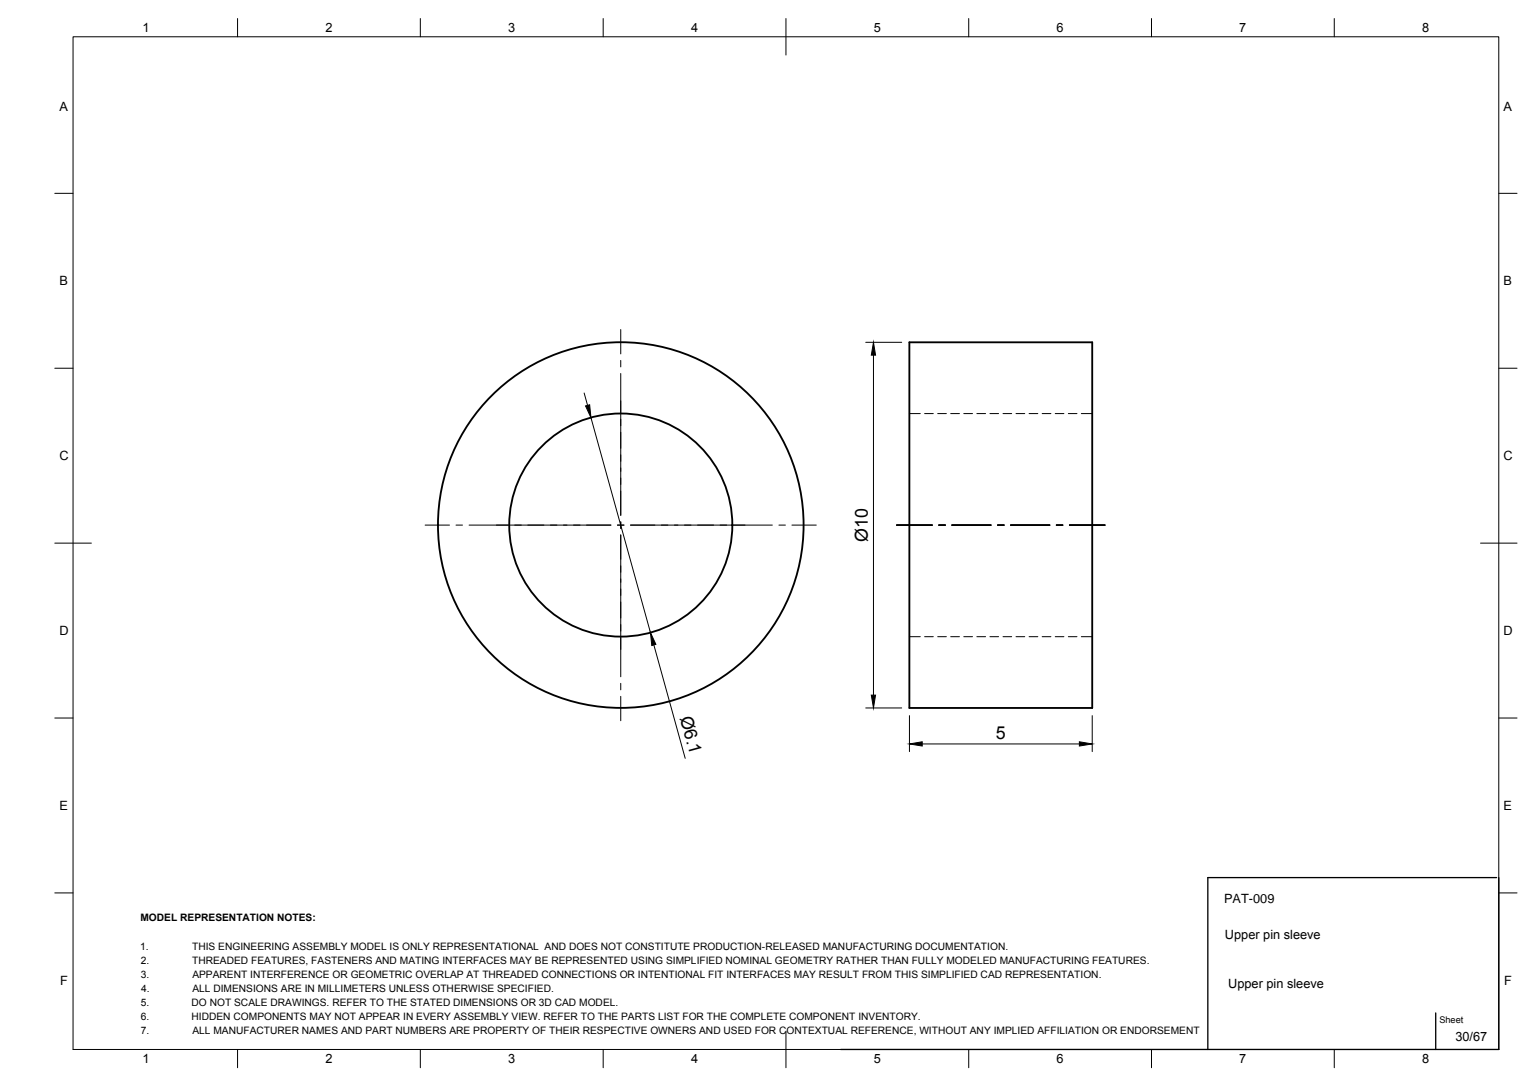
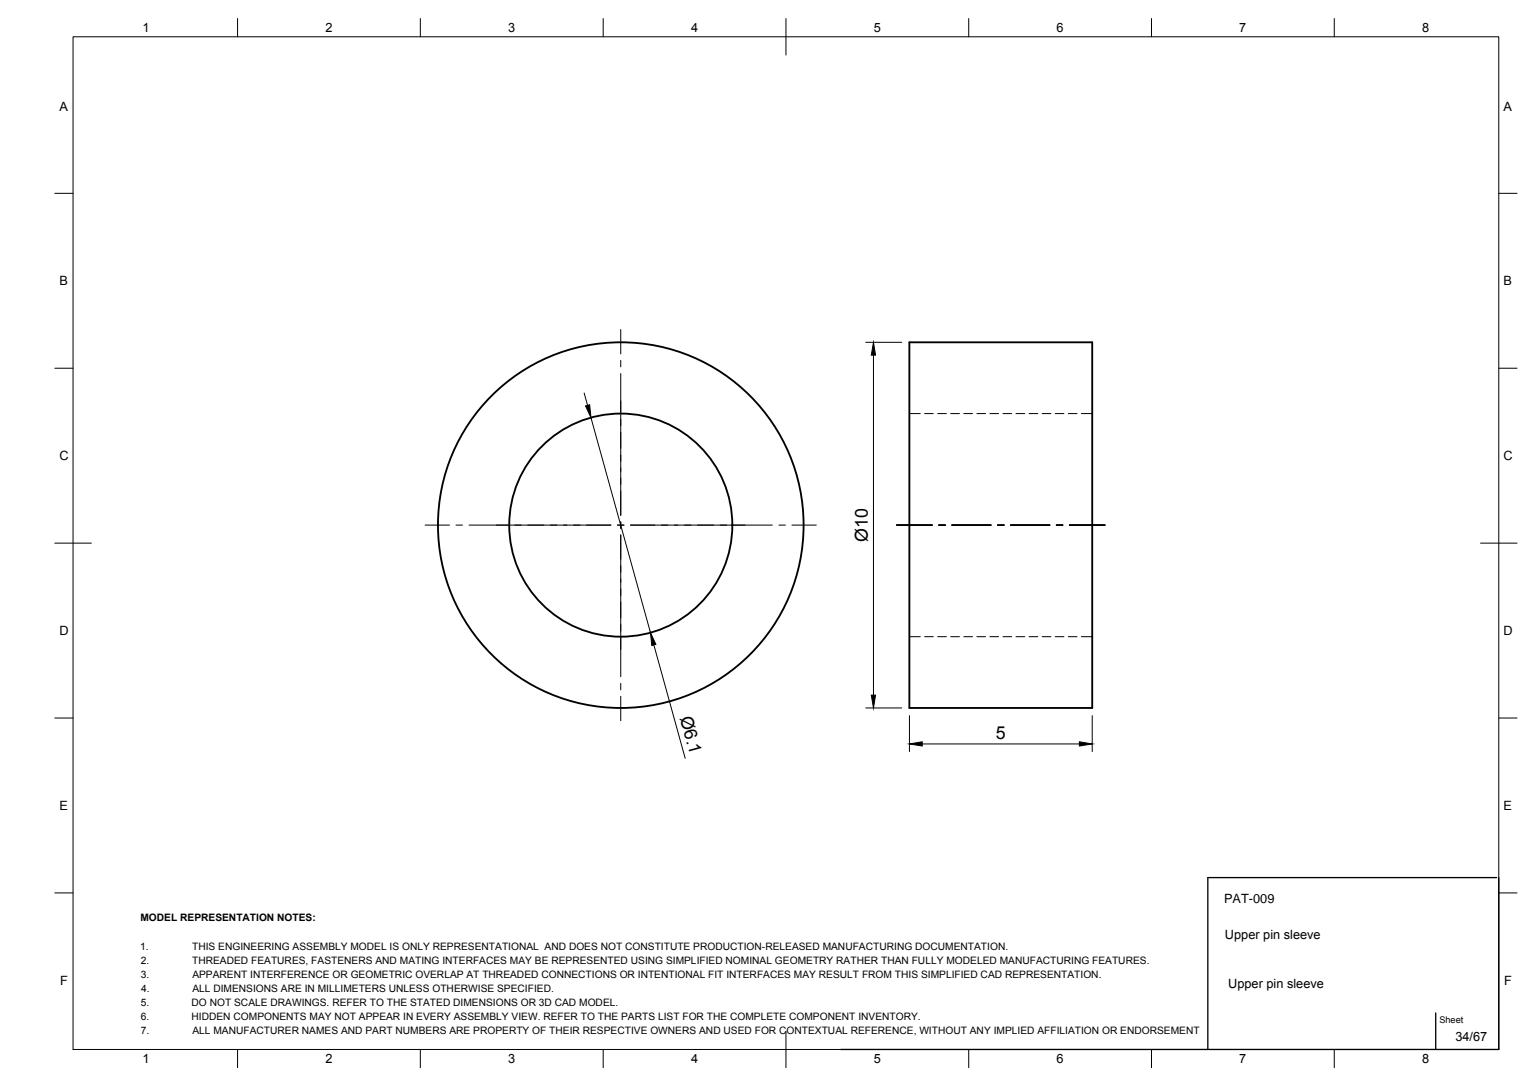
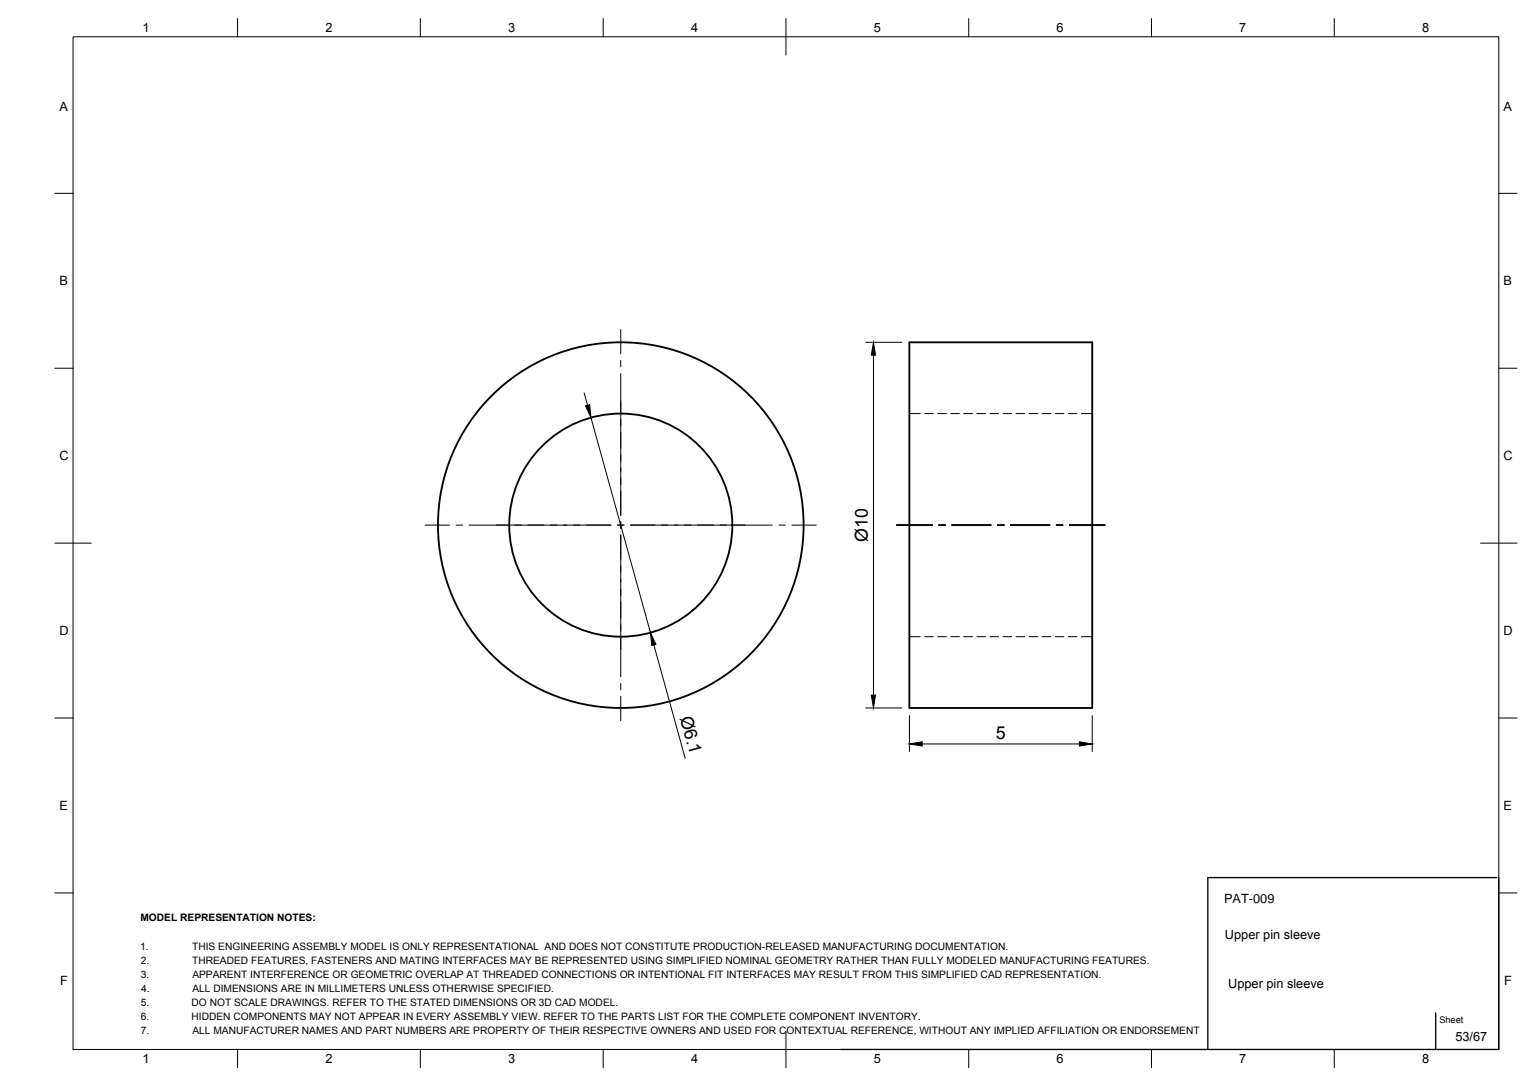
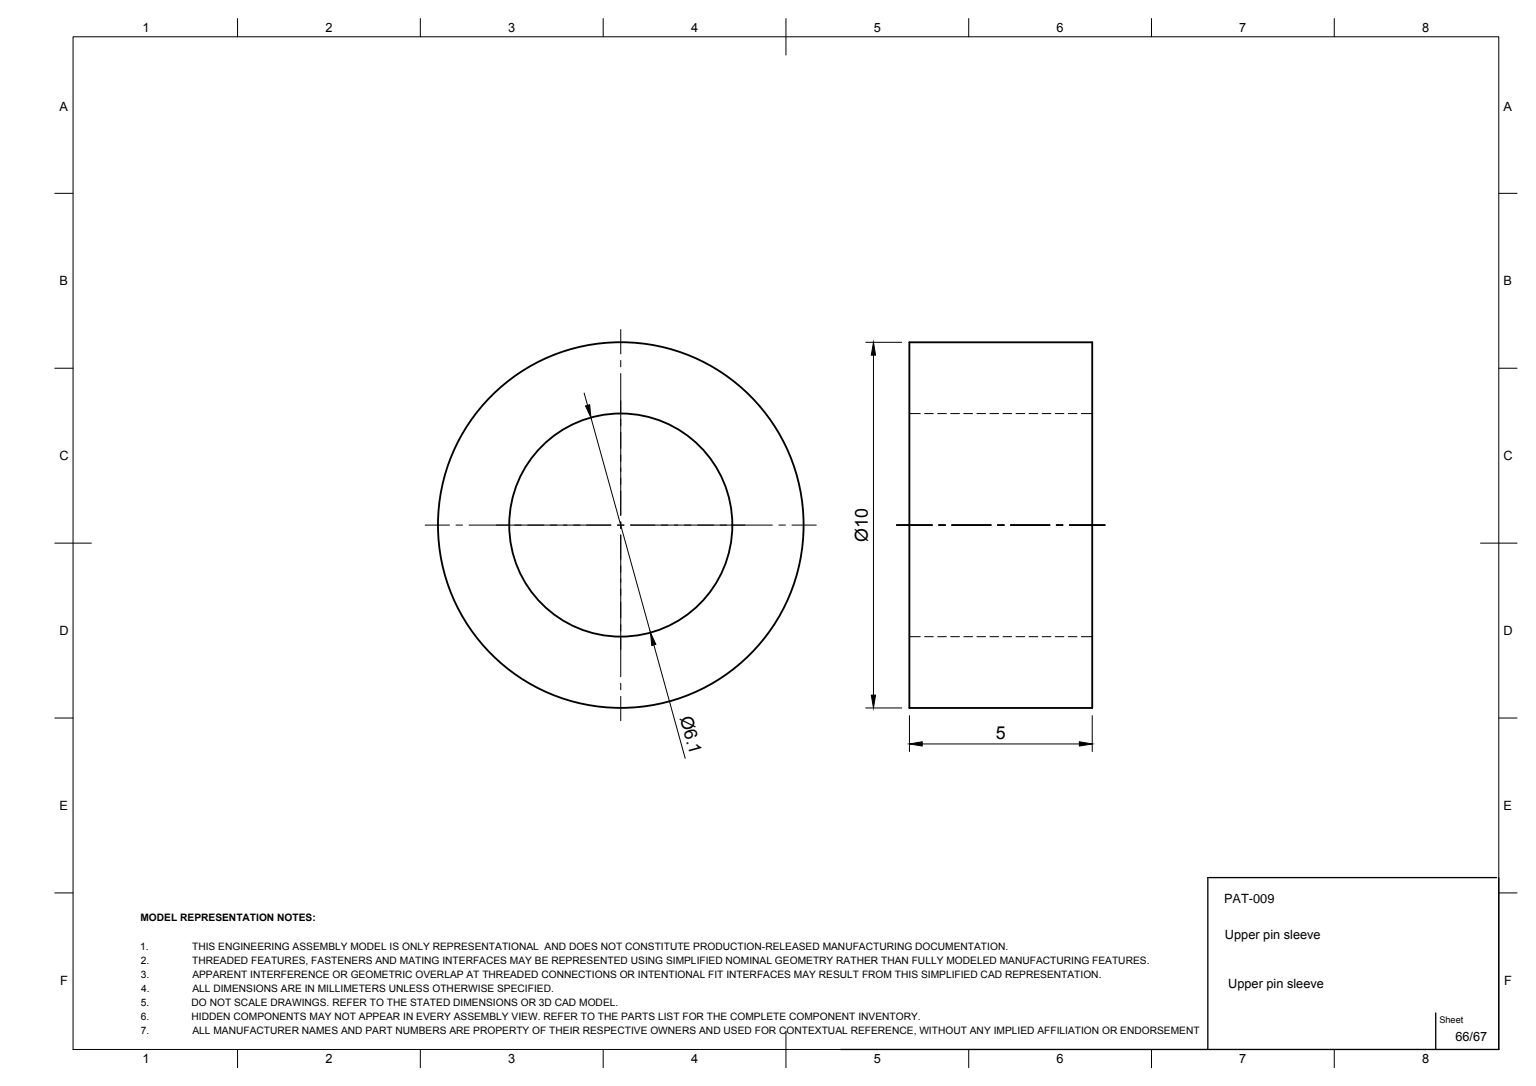
ISO-10303-21;
HEADER;
/* Generated by software containing ST-Developer
 * from STEP Tools, Inc. (www.steptools.com) 
 */

FILE_DESCRIPTION(
/* description */ ('Bell-crank linkage with push rods'),
/* implementation_level */ '2;1');

FILE_NAME(
/* name */ 'Upper pin sleeve.step',
/* time_stamp */ '2026-10-28T03:25:15-07:00',
/* author */ (''),
/* organization */ (''),
/* preprocessor_version */ 'ST-DEVELOPER v20.2',
/* originating_system */ 'Autodesk Translation Framework v15.17.0.0',
/* authorisation */ '');

FILE_SCHEMA (('AUTOMOTIVE_DESIGN { 1 0 10303 214 3 1 1 }'));
ENDSEC;

DATA;
#10=MECHANICAL_DESIGN_GEOMETRIC_PRESENTATION_REPRESENTATION('',(#635),#16678);
#519=SHAPE_REPRESENTATION_RELATIONSHIP('SRR','None',#16937,#573);
#573=ADVANCED_BREP_SHAPE_REPRESENTATION('',(#696),#16642);
#635=STYLED_ITEM('',(#17291),#696);
#696=MANIFOLD_SOLID_BREP('Body1',#8826);
#843=FACE_BOUND('',#2170,.T.);
#844=FACE_BOUND('',#2172,.T.);
#1108=PLANE('',#10059);
#1109=PLANE('',#10060);
#1527=FACE_OUTER_BOUND('',#2167,.T.);
#1528=FACE_OUTER_BOUND('',#2168,.T.);
#1529=FACE_OUTER_BOUND('',#2169,.T.);
#1530=FACE_OUTER_BOUND('',#2171,.T.);
#2167=EDGE_LOOP('',(#7141,#7142,#7143,#7144));
#2168=EDGE_LOOP('',(#7145,#7146,#7147,#7148));
#2169=EDGE_LOOP('',(#7149));
#2170=EDGE_LOOP('',(#7150));
#2171=EDGE_LOOP('',(#7151));
#2172=EDGE_LOOP('',(#7152));
#2822=LINE('',#15413,#3371);
#2823=LINE('',#15419,#3372);
#3371=VECTOR('',#12122,0.305);
#3372=VECTOR('',#12129,0.5);
#3916=CIRCLE('',#10054,0.305);
#3917=CIRCLE('',#10055,0.305);
#3918=CIRCLE('',#10057,0.5);
#3919=CIRCLE('',#10058,0.5);
#4527=VERTEX_POINT('',#15410);
#4528=VERTEX_POINT('',#15412);
#4529=VERTEX_POINT('',#15416);
#4530=VERTEX_POINT('',#15418);
#5448=EDGE_CURVE('',#4527,#4527,#3916,.T.);
#5449=EDGE_CURVE('',#4527,#4528,#2822,.T.);
#5450=EDGE_CURVE('',#4528,#4528,#3917,.T.);
#5451=EDGE_CURVE('',#4529,#4529,#3918,.T.);
#5452=EDGE_CURVE('',#4529,#4530,#2823,.T.);
#5453=EDGE_CURVE('',#4530,#4530,#3919,.T.);
#7141=ORIENTED_EDGE('',*,*,#5448,.F.);
#7142=ORIENTED_EDGE('',*,*,#5449,.T.);
#7143=ORIENTED_EDGE('',*,*,#5450,.T.);
#7144=ORIENTED_EDGE('',*,*,#5449,.F.);
#7145=ORIENTED_EDGE('',*,*,#5451,.F.);
#7146=ORIENTED_EDGE('',*,*,#5452,.T.);
#7147=ORIENTED_EDGE('',*,*,#5453,.T.);
#7148=ORIENTED_EDGE('',*,*,#5452,.F.);
#7149=ORIENTED_EDGE('',*,*,#5451,.T.);
#7150=ORIENTED_EDGE('',*,*,#5448,.T.);
#7151=ORIENTED_EDGE('',*,*,#5453,.F.);
#7152=ORIENTED_EDGE('',*,*,#5450,.F.);
#8177=CYLINDRICAL_SURFACE('',#10053,0.305);
#8178=CYLINDRICAL_SURFACE('',#10056,0.5);
#8552=ADVANCED_FACE('',(#1527),#8177,.F.);
#8553=ADVANCED_FACE('',(#1528),#8178,.T.);
#8554=ADVANCED_FACE('',(#1529,#843),#1108,.T.);
#8555=ADVANCED_FACE('',(#1530,#844),#1109,.F.);
#8826=CLOSED_SHELL('',(#8552,#8553,#8554,#8555));
#10052=AXIS2_PLACEMENT_3D('',#15408,#12116,#12117);
#10053=AXIS2_PLACEMENT_3D('',#15409,#12118,#12119);
#10054=AXIS2_PLACEMENT_3D('',#15411,#12120,#12121);
#10055=AXIS2_PLACEMENT_3D('',#15414,#12123,#12124);
#10056=AXIS2_PLACEMENT_3D('',#15415,#12125,#12126);
#10057=AXIS2_PLACEMENT_3D('',#15417,#12127,#12128);
#10058=AXIS2_PLACEMENT_3D('',#15420,#12130,#12131);
#10059=AXIS2_PLACEMENT_3D('',#15421,#12132,#12133);
#10060=AXIS2_PLACEMENT_3D('',#15422,#12134,#12135);
#12116=DIRECTION('axis',(0.,0.,1.));
#12117=DIRECTION('refdir',(1.,0.,0.));
#12118=DIRECTION('center_axis',(0.,0.,1.));
#12119=DIRECTION('ref_axis',(1.,0.,0.));
#12120=DIRECTION('center_axis',(0.,0.,-1.));
#12121=DIRECTION('ref_axis',(1.,0.,0.));
#12122=DIRECTION('',(0.,0.,-1.));
#12123=DIRECTION('center_axis',(0.,0.,-1.));
#12124=DIRECTION('ref_axis',(1.,0.,0.));
#12125=DIRECTION('center_axis',(0.,0.,1.));
#12126=DIRECTION('ref_axis',(1.,0.,0.));
#12127=DIRECTION('center_axis',(0.,0.,1.));
#12128=DIRECTION('ref_axis',(1.,0.,0.));
#12129=DIRECTION('',(0.,0.,-1.));
#12130=DIRECTION('center_axis',(0.,0.,1.));
#12131=DIRECTION('ref_axis',(1.,0.,0.));
#12132=DIRECTION('center_axis',(0.,0.,1.));
#12133=DIRECTION('ref_axis',(1.,0.,0.));
#12134=DIRECTION('center_axis',(0.,0.,1.));
#12135=DIRECTION('ref_axis',(1.,0.,0.));
#15408=CARTESIAN_POINT('',(0.,0.,0.));
#15409=CARTESIAN_POINT('Origin',(0.,2.,9.6));
#15410=CARTESIAN_POINT('',(-0.305,2.,10.1));
#15411=CARTESIAN_POINT('Origin',(0.,2.,10.1));
#15412=CARTESIAN_POINT('',(-0.305,2.,9.6));
#15413=CARTESIAN_POINT('',(-0.305,2.,9.6));
#15414=CARTESIAN_POINT('Origin',(0.,2.,9.6));
#15415=CARTESIAN_POINT('Origin',(0.,2.,9.6));
#15416=CARTESIAN_POINT('',(-0.5,2.,10.1));
#15417=CARTESIAN_POINT('Origin',(0.,2.,10.1));
#15418=CARTESIAN_POINT('',(-0.5,2.,9.6));
#15419=CARTESIAN_POINT('',(-0.5,2.,9.6));
#15420=CARTESIAN_POINT('Origin',(0.,2.,9.6));
#15421=CARTESIAN_POINT('Origin',(0.,2.,10.1));
#15422=CARTESIAN_POINT('Origin',(0.,2.,9.6));
#16578=UNCERTAINTY_MEASURE_WITH_UNIT(LENGTH_MEASURE(0.001),#16679,
'DISTANCE_ACCURACY_VALUE',
'Maximum model space distance between geometric entities at asserted c
onnectivities');
#16614=UNCERTAINTY_MEASURE_WITH_UNIT(LENGTH_MEASURE(0.001),#16679,
'DISTANCE_ACCURACY_VALUE',
'Maximum model space distance between geometric entities at asserted c
onnectivities');
#16642=(
GEOMETRIC_REPRESENTATION_CONTEXT(3)
GLOBAL_UNCERTAINTY_ASSIGNED_CONTEXT((#16578))
GLOBAL_UNIT_ASSIGNED_CONTEXT((#16679,#16681,#16682))
REPRESENTATION_CONTEXT('','3D')
);
#16678=(
GEOMETRIC_REPRESENTATION_CONTEXT(3)
GLOBAL_UNCERTAINTY_ASSIGNED_CONTEXT((#16614))
GLOBAL_UNIT_ASSIGNED_CONTEXT((#16679,#16681,#16682))
REPRESENTATION_CONTEXT('','3D')
);
#16679=(
LENGTH_UNIT()
NAMED_UNIT(*)
SI_UNIT(.CENTI.,.METRE.)
);
#16681=(
NAMED_UNIT(*)
PLANE_ANGLE_UNIT()
SI_UNIT($,.RADIAN.)
);
#16682=(
NAMED_UNIT(*)
SI_UNIT($,.STERADIAN.)
SOLID_ANGLE_UNIT()
);
#16710=SHAPE_DEFINITION_REPRESENTATION(#16778,#16937);
#16778=PRODUCT_DEFINITION_SHAPE('',$,#17001);
#16937=SHAPE_REPRESENTATION('',(#10052),#16642);
#16973=PRODUCT_DEFINITION_CONTEXT('part definition',#17164,'design');
#17001=PRODUCT_DEFINITION('Upper pin sleeve','Upper pin sleeve',#17064,
#16973);
#17064=PRODUCT_DEFINITION_FORMATION('',$,#17193);
#17164=APPLICATION_CONTEXT(
'Core Data for Automotive Mechanical Design Process');
#17165=PRODUCT_CONTEXT('part definition',#17164,'mechanical');
#17193=PRODUCT('Upper pin sleeve','Upper pin sleeve','Upper pin sleeve',
(#17165));
#17285=COLOUR_RGB('Grey',0.48,0.52,0.57);
#17286=FILL_AREA_STYLE_COLOUR('',#17285);
#17287=FILL_AREA_STYLE('',(#17286));
#17288=SURFACE_STYLE_FILL_AREA(#17287);
#17289=SURFACE_SIDE_STYLE('',(#17288));
#17290=SURFACE_STYLE_USAGE(.BOTH.,#17289);
#17291=PRESENTATION_STYLE_ASSIGNMENT((#17290));
ENDSEC;
END-ISO-10303-21;
